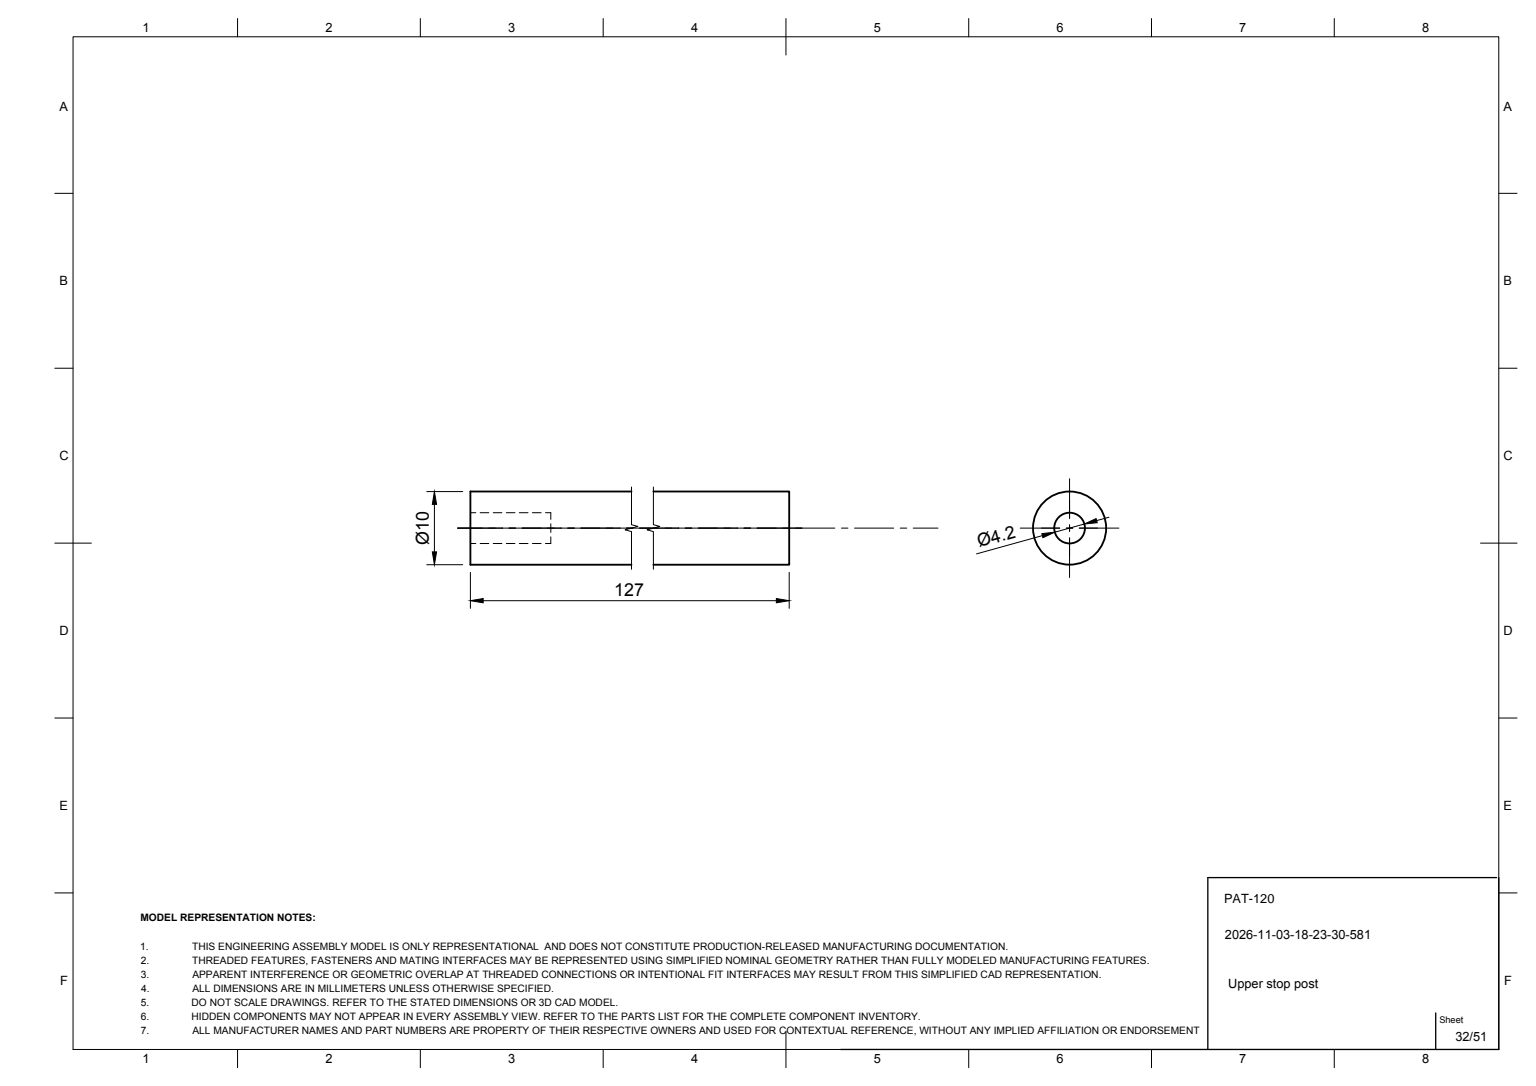
ISO-10303-21;
HEADER;
/* Generated by software containing ST-Developer
 * from STEP Tools, Inc. (www.steptools.com) 
 */

FILE_DESCRIPTION(
/* description */ ('Vibration shaker table dummy'),
/* implementation_level */ '2;1');

FILE_NAME(
/* name */ 'Upper stop post.step',
/* time_stamp */ '2026-10-27T10:55:14-07:00',
/* author */ (''),
/* organization */ (''),
/* preprocessor_version */ 'ST-DEVELOPER v20.2',
/* originating_system */ 'Autodesk Translation Framework v15.17.0.0',
/* authorisation */ '');

FILE_SCHEMA (('AUTOMOTIVE_DESIGN { 1 0 10303 214 3 1 1 }'));
ENDSEC;

DATA;
#10=MECHANICAL_DESIGN_GEOMETRIC_PRESENTATION_REPRESENTATION('',(#713),#22394);
#621=SHAPE_REPRESENTATION_RELATIONSHIP('SRR','None',#22667,#667);
#667=ADVANCED_BREP_SHAPE_REPRESENTATION('',(#759),#22373);
#713=STYLED_ITEM('',(#22975),#759);
#759=MANIFOLD_SOLID_BREP('Body1',#9231);
#944=FACE_BOUND('',#2280,.T.);
#1217=PLANE('',#10295);
#1218=PLANE('',#10299);
#1219=PLANE('',#10300);
#1609=FACE_OUTER_BOUND('',#2276,.T.);
#1610=FACE_OUTER_BOUND('',#2277,.T.);
#1611=FACE_OUTER_BOUND('',#2278,.T.);
#1612=FACE_OUTER_BOUND('',#2279,.T.);
#1613=FACE_OUTER_BOUND('',#2281,.T.);
#2276=EDGE_LOOP('',(#7440,#7441,#7442,#7443));
#2277=EDGE_LOOP('',(#7444));
#2278=EDGE_LOOP('',(#7445,#7446,#7447,#7448));
#2279=EDGE_LOOP('',(#7449));
#2280=EDGE_LOOP('',(#7450));
#2281=EDGE_LOOP('',(#7451));
#2977=LINE('',#21024,#3596);
#2978=LINE('',#21031,#3597);
#3596=VECTOR('',#12373,0.21);
#3597=VECTOR('',#12382,0.5);
#4098=CIRCLE('',#10293,0.21);
#4099=CIRCLE('',#10294,0.21);
#4100=CIRCLE('',#10297,0.5);
#4101=CIRCLE('',#10298,0.5);
#4765=VERTEX_POINT('',#21021);
#4766=VERTEX_POINT('',#21023);
#4767=VERTEX_POINT('',#21028);
#4768=VERTEX_POINT('',#21030);
#5713=EDGE_CURVE('',#4765,#4765,#4098,.T.);
#5714=EDGE_CURVE('',#4765,#4766,#2977,.T.);
#5715=EDGE_CURVE('',#4766,#4766,#4099,.T.);
#5716=EDGE_CURVE('',#4767,#4767,#4100,.T.);
#5717=EDGE_CURVE('',#4767,#4768,#2978,.T.);
#5718=EDGE_CURVE('',#4768,#4768,#4101,.T.);
#7440=ORIENTED_EDGE('',*,*,#5713,.F.);
#7441=ORIENTED_EDGE('',*,*,#5714,.T.);
#7442=ORIENTED_EDGE('',*,*,#5715,.F.);
#7443=ORIENTED_EDGE('',*,*,#5714,.F.);
#7444=ORIENTED_EDGE('',*,*,#5713,.T.);
#7445=ORIENTED_EDGE('',*,*,#5716,.F.);
#7446=ORIENTED_EDGE('',*,*,#5717,.T.);
#7447=ORIENTED_EDGE('',*,*,#5718,.T.);
#7448=ORIENTED_EDGE('',*,*,#5717,.F.);
#7449=ORIENTED_EDGE('',*,*,#5716,.T.);
#7450=ORIENTED_EDGE('',*,*,#5715,.T.);
#7451=ORIENTED_EDGE('',*,*,#5718,.F.);
#8613=CYLINDRICAL_SURFACE('',#10292,0.21);
#8614=CYLINDRICAL_SURFACE('',#10296,0.5);
#8974=ADVANCED_FACE('',(#1609),#8613,.F.);
#8975=ADVANCED_FACE('',(#1610),#1217,.T.);
#8976=ADVANCED_FACE('',(#1611),#8614,.T.);
#8977=ADVANCED_FACE('',(#1612,#944),#1218,.T.);
#8978=ADVANCED_FACE('',(#1613),#1219,.F.);
#9231=CLOSED_SHELL('',(#8974,#8975,#8976,#8977,#8978));
#10291=AXIS2_PLACEMENT_3D('',#21019,#12367,#12368);
#10292=AXIS2_PLACEMENT_3D('',#21020,#12369,#12370);
#10293=AXIS2_PLACEMENT_3D('',#21022,#12371,#12372);
#10294=AXIS2_PLACEMENT_3D('',#21025,#12374,#12375);
#10295=AXIS2_PLACEMENT_3D('',#21026,#12376,#12377);
#10296=AXIS2_PLACEMENT_3D('',#21027,#12378,#12379);
#10297=AXIS2_PLACEMENT_3D('',#21029,#12380,#12381);
#10298=AXIS2_PLACEMENT_3D('',#21032,#12383,#12384);
#10299=AXIS2_PLACEMENT_3D('',#21033,#12385,#12386);
#10300=AXIS2_PLACEMENT_3D('',#21034,#12387,#12388);
#12367=DIRECTION('axis',(0.,0.,1.));
#12368=DIRECTION('refdir',(1.,0.,0.));
#12369=DIRECTION('center_axis',(0.,0.,1.));
#12370=DIRECTION('ref_axis',(1.,0.,0.));
#12371=DIRECTION('center_axis',(0.,0.,1.));
#12372=DIRECTION('ref_axis',(1.,0.,0.));
#12373=DIRECTION('',(0.,0.,1.));
#12374=DIRECTION('center_axis',(0.,0.,-1.));
#12375=DIRECTION('ref_axis',(1.,0.,0.));
#12376=DIRECTION('center_axis',(0.,0.,1.));
#12377=DIRECTION('ref_axis',(1.,0.,0.));
#12378=DIRECTION('center_axis',(0.,0.,1.));
#12379=DIRECTION('ref_axis',(1.,0.,0.));
#12380=DIRECTION('center_axis',(0.,0.,1.));
#12381=DIRECTION('ref_axis',(1.,0.,0.));
#12382=DIRECTION('',(0.,0.,-1.));
#12383=DIRECTION('center_axis',(0.,0.,1.));
#12384=DIRECTION('ref_axis',(1.,0.,0.));
#12385=DIRECTION('center_axis',(0.,0.,1.));
#12386=DIRECTION('ref_axis',(1.,0.,0.));
#12387=DIRECTION('center_axis',(0.,0.,1.));
#12388=DIRECTION('ref_axis',(1.,0.,0.));
#21019=CARTESIAN_POINT('',(0.,0.,0.));
#21020=CARTESIAN_POINT('Origin',(0.,-6.,29.4));
#21021=CARTESIAN_POINT('',(-0.21,-6.,29.4));
#21022=CARTESIAN_POINT('Origin',(0.,-6.,29.4));
#21023=CARTESIAN_POINT('',(-0.21,-6.,30.5));
#21024=CARTESIAN_POINT('',(-0.21,-6.,29.4));
#21025=CARTESIAN_POINT('Origin',(0.,-6.,30.5));
#21026=CARTESIAN_POINT('Origin',(0.,-6.,29.4));
#21027=CARTESIAN_POINT('Origin',(0.,-6.,17.8));
#21028=CARTESIAN_POINT('',(-0.5,-6.,30.5));
#21029=CARTESIAN_POINT('Origin',(0.,-6.,30.5));
#21030=CARTESIAN_POINT('',(-0.5,-6.,17.8));
#21031=CARTESIAN_POINT('',(-0.5,-6.,17.8));
#21032=CARTESIAN_POINT('Origin',(0.,-6.,17.8));
#21033=CARTESIAN_POINT('Origin',(0.,-6.,30.5));
#21034=CARTESIAN_POINT('Origin',(0.,-6.,17.8));
#22322=UNCERTAINTY_MEASURE_WITH_UNIT(LENGTH_MEASURE(0.001),#22395,
'DISTANCE_ACCURACY_VALUE',
'Maximum model space distance between geometric entities at asserted c
onnectivities');
#22343=UNCERTAINTY_MEASURE_WITH_UNIT(LENGTH_MEASURE(0.001),#22395,
'DISTANCE_ACCURACY_VALUE',
'Maximum model space distance between geometric entities at asserted c
onnectivities');
#22373=(
GEOMETRIC_REPRESENTATION_CONTEXT(3)
GLOBAL_UNCERTAINTY_ASSIGNED_CONTEXT((#22322))
GLOBAL_UNIT_ASSIGNED_CONTEXT((#22395,#22397,#22398))
REPRESENTATION_CONTEXT('','3D')
);
#22394=(
GEOMETRIC_REPRESENTATION_CONTEXT(3)
GLOBAL_UNCERTAINTY_ASSIGNED_CONTEXT((#22343))
GLOBAL_UNIT_ASSIGNED_CONTEXT((#22395,#22397,#22398))
REPRESENTATION_CONTEXT('','3D')
);
#22395=(
LENGTH_UNIT()
NAMED_UNIT(*)
SI_UNIT(.CENTI.,.METRE.)
);
#22397=(
NAMED_UNIT(*)
PLANE_ANGLE_UNIT()
SI_UNIT($,.RADIAN.)
);
#22398=(
NAMED_UNIT(*)
SI_UNIT($,.STERADIAN.)
SOLID_ANGLE_UNIT()
);
#22428=SHAPE_DEFINITION_REPRESENTATION(#22478,#22667);
#22478=PRODUCT_DEFINITION_SHAPE('',$,#22718);
#22667=SHAPE_REPRESENTATION('',(#10291),#22373);
#22688=PRODUCT_DEFINITION_CONTEXT('part definition',#22840,'design');
#22718=PRODUCT_DEFINITION('Upper stop post','Upper stop post',#22768,#22688);
#22768=PRODUCT_DEFINITION_FORMATION('',$,#22871);
#22840=APPLICATION_CONTEXT(
'Core Data for Automotive Mechanical Design Process');
#22841=PRODUCT_CONTEXT('part definition',#22840,'mechanical');
#22871=PRODUCT('Upper stop post','Upper stop post','Upper stop post',(#22841));
#22969=COLOUR_RGB('Off White',0.89,0.88,0.83);
#22970=FILL_AREA_STYLE_COLOUR('',#22969);
#22971=FILL_AREA_STYLE('',(#22970));
#22972=SURFACE_STYLE_FILL_AREA(#22971);
#22973=SURFACE_SIDE_STYLE('',(#22972));
#22974=SURFACE_STYLE_USAGE(.BOTH.,#22973);
#22975=PRESENTATION_STYLE_ASSIGNMENT((#22974));
ENDSEC;
END-ISO-10303-21;
